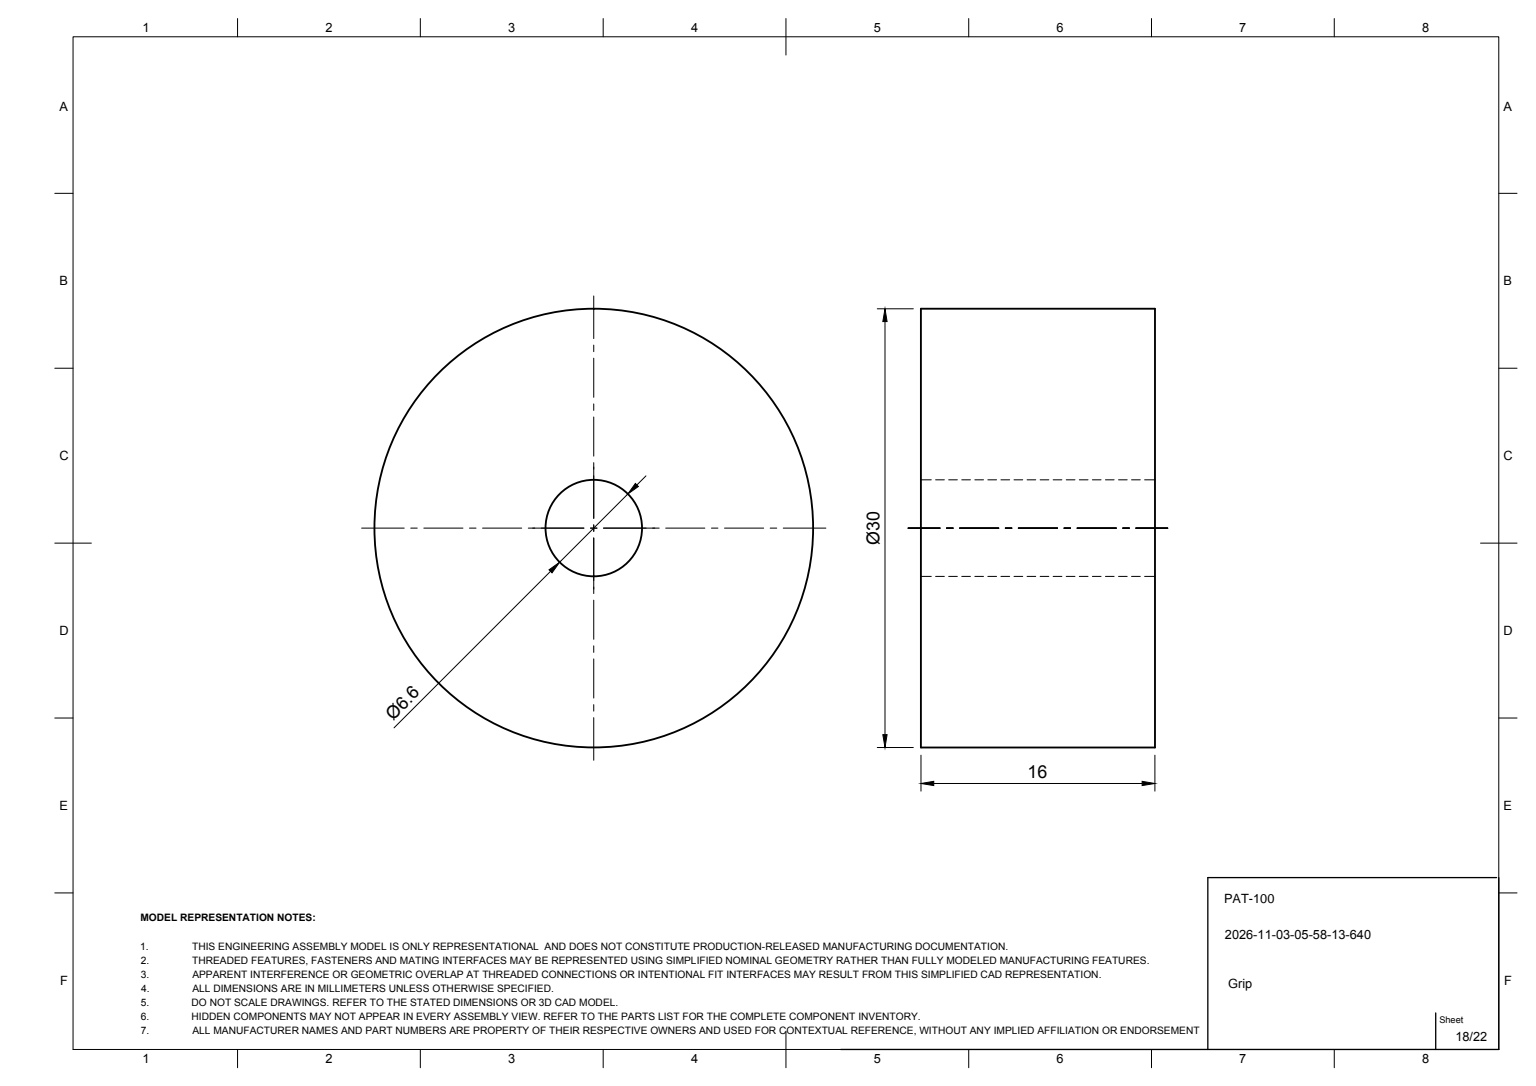
ISO-10303-21;
HEADER;
/* Generated by software containing ST-Developer
 * from STEP Tools, Inc. (www.steptools.com) 
 */

FILE_DESCRIPTION(
/* description */ (''),
/* implementation_level */ '2;1');

FILE_NAME(
/* name */ 'Grip.step',
/* time_stamp */ '2026-10-29T16:43:51-07:00',
/* author */ (''),
/* organization */ (''),
/* preprocessor_version */ 'ST-DEVELOPER v20.2',
/* originating_system */ 'Autodesk Translation Framework v15.17.0.0',
/* authorisation */ '');

FILE_SCHEMA (('AUTOMOTIVE_DESIGN { 1 0 10303 214 3 1 1 }'));
ENDSEC;

DATA;
#10=MECHANICAL_DESIGN_GEOMETRIC_PRESENTATION_REPRESENTATION('',(#385),#10292);
#339=SHAPE_REPRESENTATION_RELATIONSHIP('SRR','None',#10437,#362);
#362=ADVANCED_BREP_SHAPE_REPRESENTATION('',(#404),#10289);
#385=STYLED_ITEM('',(#10635),#404);
#404=MANIFOLD_SOLID_BREP('Body1',#5031);
#526=FACE_BOUND('',#1384,.T.);
#527=FACE_BOUND('',#1386,.T.);
#695=PLANE('',#5804);
#696=PLANE('',#5805);
#973=FACE_OUTER_BOUND('',#1381,.T.);
#974=FACE_OUTER_BOUND('',#1382,.T.);
#975=FACE_OUTER_BOUND('',#1383,.T.);
#976=FACE_OUTER_BOUND('',#1385,.T.);
#1381=EDGE_LOOP('',(#4549,#4550,#4551,#4552));
#1382=EDGE_LOOP('',(#4553,#4554,#4555,#4556));
#1383=EDGE_LOOP('',(#4557));
#1384=EDGE_LOOP('',(#4558));
#1385=EDGE_LOOP('',(#4559));
#1386=EDGE_LOOP('',(#4560));
#1775=LINE('',#10119,#2167);
#1776=LINE('',#10125,#2168);
#2167=VECTOR('',#7250,0.33);
#2168=VECTOR('',#7257,1.5);
#2378=CIRCLE('',#5799,0.33);
#2379=CIRCLE('',#5800,0.33);
#2380=CIRCLE('',#5802,1.5);
#2381=CIRCLE('',#5803,1.5);
#2767=VERTEX_POINT('',#10116);
#2768=VERTEX_POINT('',#10118);
#2769=VERTEX_POINT('',#10122);
#2770=VERTEX_POINT('',#10124);
#3365=EDGE_CURVE('',#2767,#2767,#2378,.T.);
#3366=EDGE_CURVE('',#2767,#2768,#1775,.T.);
#3367=EDGE_CURVE('',#2768,#2768,#2379,.T.);
#3368=EDGE_CURVE('',#2769,#2769,#2380,.T.);
#3369=EDGE_CURVE('',#2769,#2770,#1776,.T.);
#3370=EDGE_CURVE('',#2770,#2770,#2381,.T.);
#4549=ORIENTED_EDGE('',*,*,#3365,.F.);
#4550=ORIENTED_EDGE('',*,*,#3366,.T.);
#4551=ORIENTED_EDGE('',*,*,#3367,.T.);
#4552=ORIENTED_EDGE('',*,*,#3366,.F.);
#4553=ORIENTED_EDGE('',*,*,#3368,.F.);
#4554=ORIENTED_EDGE('',*,*,#3369,.T.);
#4555=ORIENTED_EDGE('',*,*,#3370,.T.);
#4556=ORIENTED_EDGE('',*,*,#3369,.F.);
#4557=ORIENTED_EDGE('',*,*,#3368,.T.);
#4558=ORIENTED_EDGE('',*,*,#3365,.T.);
#4559=ORIENTED_EDGE('',*,*,#3370,.F.);
#4560=ORIENTED_EDGE('',*,*,#3367,.F.);
#4713=CYLINDRICAL_SURFACE('',#5798,0.33);
#4714=CYLINDRICAL_SURFACE('',#5801,1.5);
#4982=ADVANCED_FACE('',(#973),#4713,.F.);
#4983=ADVANCED_FACE('',(#974),#4714,.T.);
#4984=ADVANCED_FACE('',(#975,#526),#695,.T.);
#4985=ADVANCED_FACE('',(#976,#527),#696,.F.);
#5031=CLOSED_SHELL('',(#4982,#4983,#4984,#4985));
#5797=AXIS2_PLACEMENT_3D('',#10114,#7244,#7245);
#5798=AXIS2_PLACEMENT_3D('',#10115,#7246,#7247);
#5799=AXIS2_PLACEMENT_3D('',#10117,#7248,#7249);
#5800=AXIS2_PLACEMENT_3D('',#10120,#7251,#7252);
#5801=AXIS2_PLACEMENT_3D('',#10121,#7253,#7254);
#5802=AXIS2_PLACEMENT_3D('',#10123,#7255,#7256);
#5803=AXIS2_PLACEMENT_3D('',#10126,#7258,#7259);
#5804=AXIS2_PLACEMENT_3D('',#10127,#7260,#7261);
#5805=AXIS2_PLACEMENT_3D('',#10128,#7262,#7263);
#7244=DIRECTION('axis',(0.,0.,1.));
#7245=DIRECTION('refdir',(1.,0.,0.));
#7246=DIRECTION('center_axis',(0.,0.,1.));
#7247=DIRECTION('ref_axis',(1.,0.,0.));
#7248=DIRECTION('center_axis',(0.,0.,-1.));
#7249=DIRECTION('ref_axis',(1.,0.,0.));
#7250=DIRECTION('',(0.,0.,-1.));
#7251=DIRECTION('center_axis',(0.,0.,-1.));
#7252=DIRECTION('ref_axis',(1.,0.,0.));
#7253=DIRECTION('center_axis',(0.,0.,1.));
#7254=DIRECTION('ref_axis',(1.,0.,0.));
#7255=DIRECTION('center_axis',(0.,0.,1.));
#7256=DIRECTION('ref_axis',(1.,0.,0.));
#7257=DIRECTION('',(0.,0.,-1.));
#7258=DIRECTION('center_axis',(0.,0.,1.));
#7259=DIRECTION('ref_axis',(1.,0.,0.));
#7260=DIRECTION('center_axis',(0.,0.,1.));
#7261=DIRECTION('ref_axis',(1.,0.,0.));
#7262=DIRECTION('center_axis',(0.,0.,1.));
#7263=DIRECTION('ref_axis',(1.,0.,0.));
#10114=CARTESIAN_POINT('',(0.,0.,0.));
#10115=CARTESIAN_POINT('Origin',(15.,0.,6.6));
#10116=CARTESIAN_POINT('',(14.67,-4.04133443718627E-17,8.2));
#10117=CARTESIAN_POINT('Origin',(15.,0.,8.2));
#10118=CARTESIAN_POINT('',(14.67,-4.04133443718627E-17,6.6));
#10119=CARTESIAN_POINT('',(14.67,-4.04133443718627E-17,6.6));
#10120=CARTESIAN_POINT('Origin',(15.,0.,6.6));
#10121=CARTESIAN_POINT('Origin',(15.,0.,6.6));
#10122=CARTESIAN_POINT('',(13.5,-1.83697019872103E-16,8.2));
#10123=CARTESIAN_POINT('Origin',(15.,0.,8.2));
#10124=CARTESIAN_POINT('',(13.5,-1.83697019872103E-16,6.6));
#10125=CARTESIAN_POINT('',(13.5,-1.83697019872103E-16,6.6));
#10126=CARTESIAN_POINT('Origin',(15.,0.,6.6));
#10127=CARTESIAN_POINT('Origin',(15.,0.,8.2));
#10128=CARTESIAN_POINT('Origin',(15.,0.,6.6));
#10261=UNCERTAINTY_MEASURE_WITH_UNIT(LENGTH_MEASURE(0.001),#10293,
'DISTANCE_ACCURACY_VALUE',
'Maximum model space distance between geometric entities at asserted c
onnectivities');
#10264=UNCERTAINTY_MEASURE_WITH_UNIT(LENGTH_MEASURE(0.001),#10293,
'DISTANCE_ACCURACY_VALUE',
'Maximum model space distance between geometric entities at asserted c
onnectivities');
#10289=(
GEOMETRIC_REPRESENTATION_CONTEXT(3)
GLOBAL_UNCERTAINTY_ASSIGNED_CONTEXT((#10261))
GLOBAL_UNIT_ASSIGNED_CONTEXT((#10293,#10295,#10296))
REPRESENTATION_CONTEXT('','3D')
);
#10292=(
GEOMETRIC_REPRESENTATION_CONTEXT(3)
GLOBAL_UNCERTAINTY_ASSIGNED_CONTEXT((#10264))
GLOBAL_UNIT_ASSIGNED_CONTEXT((#10293,#10295,#10296))
REPRESENTATION_CONTEXT('','3D')
);
#10293=(
LENGTH_UNIT()
NAMED_UNIT(*)
SI_UNIT(.CENTI.,.METRE.)
);
#10295=(
NAMED_UNIT(*)
PLANE_ANGLE_UNIT()
SI_UNIT($,.RADIAN.)
);
#10296=(
NAMED_UNIT(*)
SI_UNIT($,.STERADIAN.)
SOLID_ANGLE_UNIT()
);
#10321=SHAPE_DEFINITION_REPRESENTATION(#10387,#10437);
#10387=PRODUCT_DEFINITION_SHAPE('',$,#10465);
#10437=SHAPE_REPRESENTATION('',(#5797),#10289);
#10440=PRODUCT_DEFINITION_CONTEXT('part definition',#10523,'design');
#10465=PRODUCT_DEFINITION('Grip','Grip',#10492,#10440);
#10492=PRODUCT_DEFINITION_FORMATION('',$,#10549);
#10523=APPLICATION_CONTEXT(
'Core Data for Automotive Mechanical Design Process');
#10524=PRODUCT_CONTEXT('part definition',#10523,'mechanical');
#10549=PRODUCT('Grip','Grip','Grip',(#10524));
#10629=COLOUR_RGB('Black',0.12,0.14,0.17);
#10630=FILL_AREA_STYLE_COLOUR('',#10629);
#10631=FILL_AREA_STYLE('',(#10630));
#10632=SURFACE_STYLE_FILL_AREA(#10631);
#10633=SURFACE_SIDE_STYLE('',(#10632));
#10634=SURFACE_STYLE_USAGE(.BOTH.,#10633);
#10635=PRESENTATION_STYLE_ASSIGNMENT((#10634));
ENDSEC;
END-ISO-10303-21;
